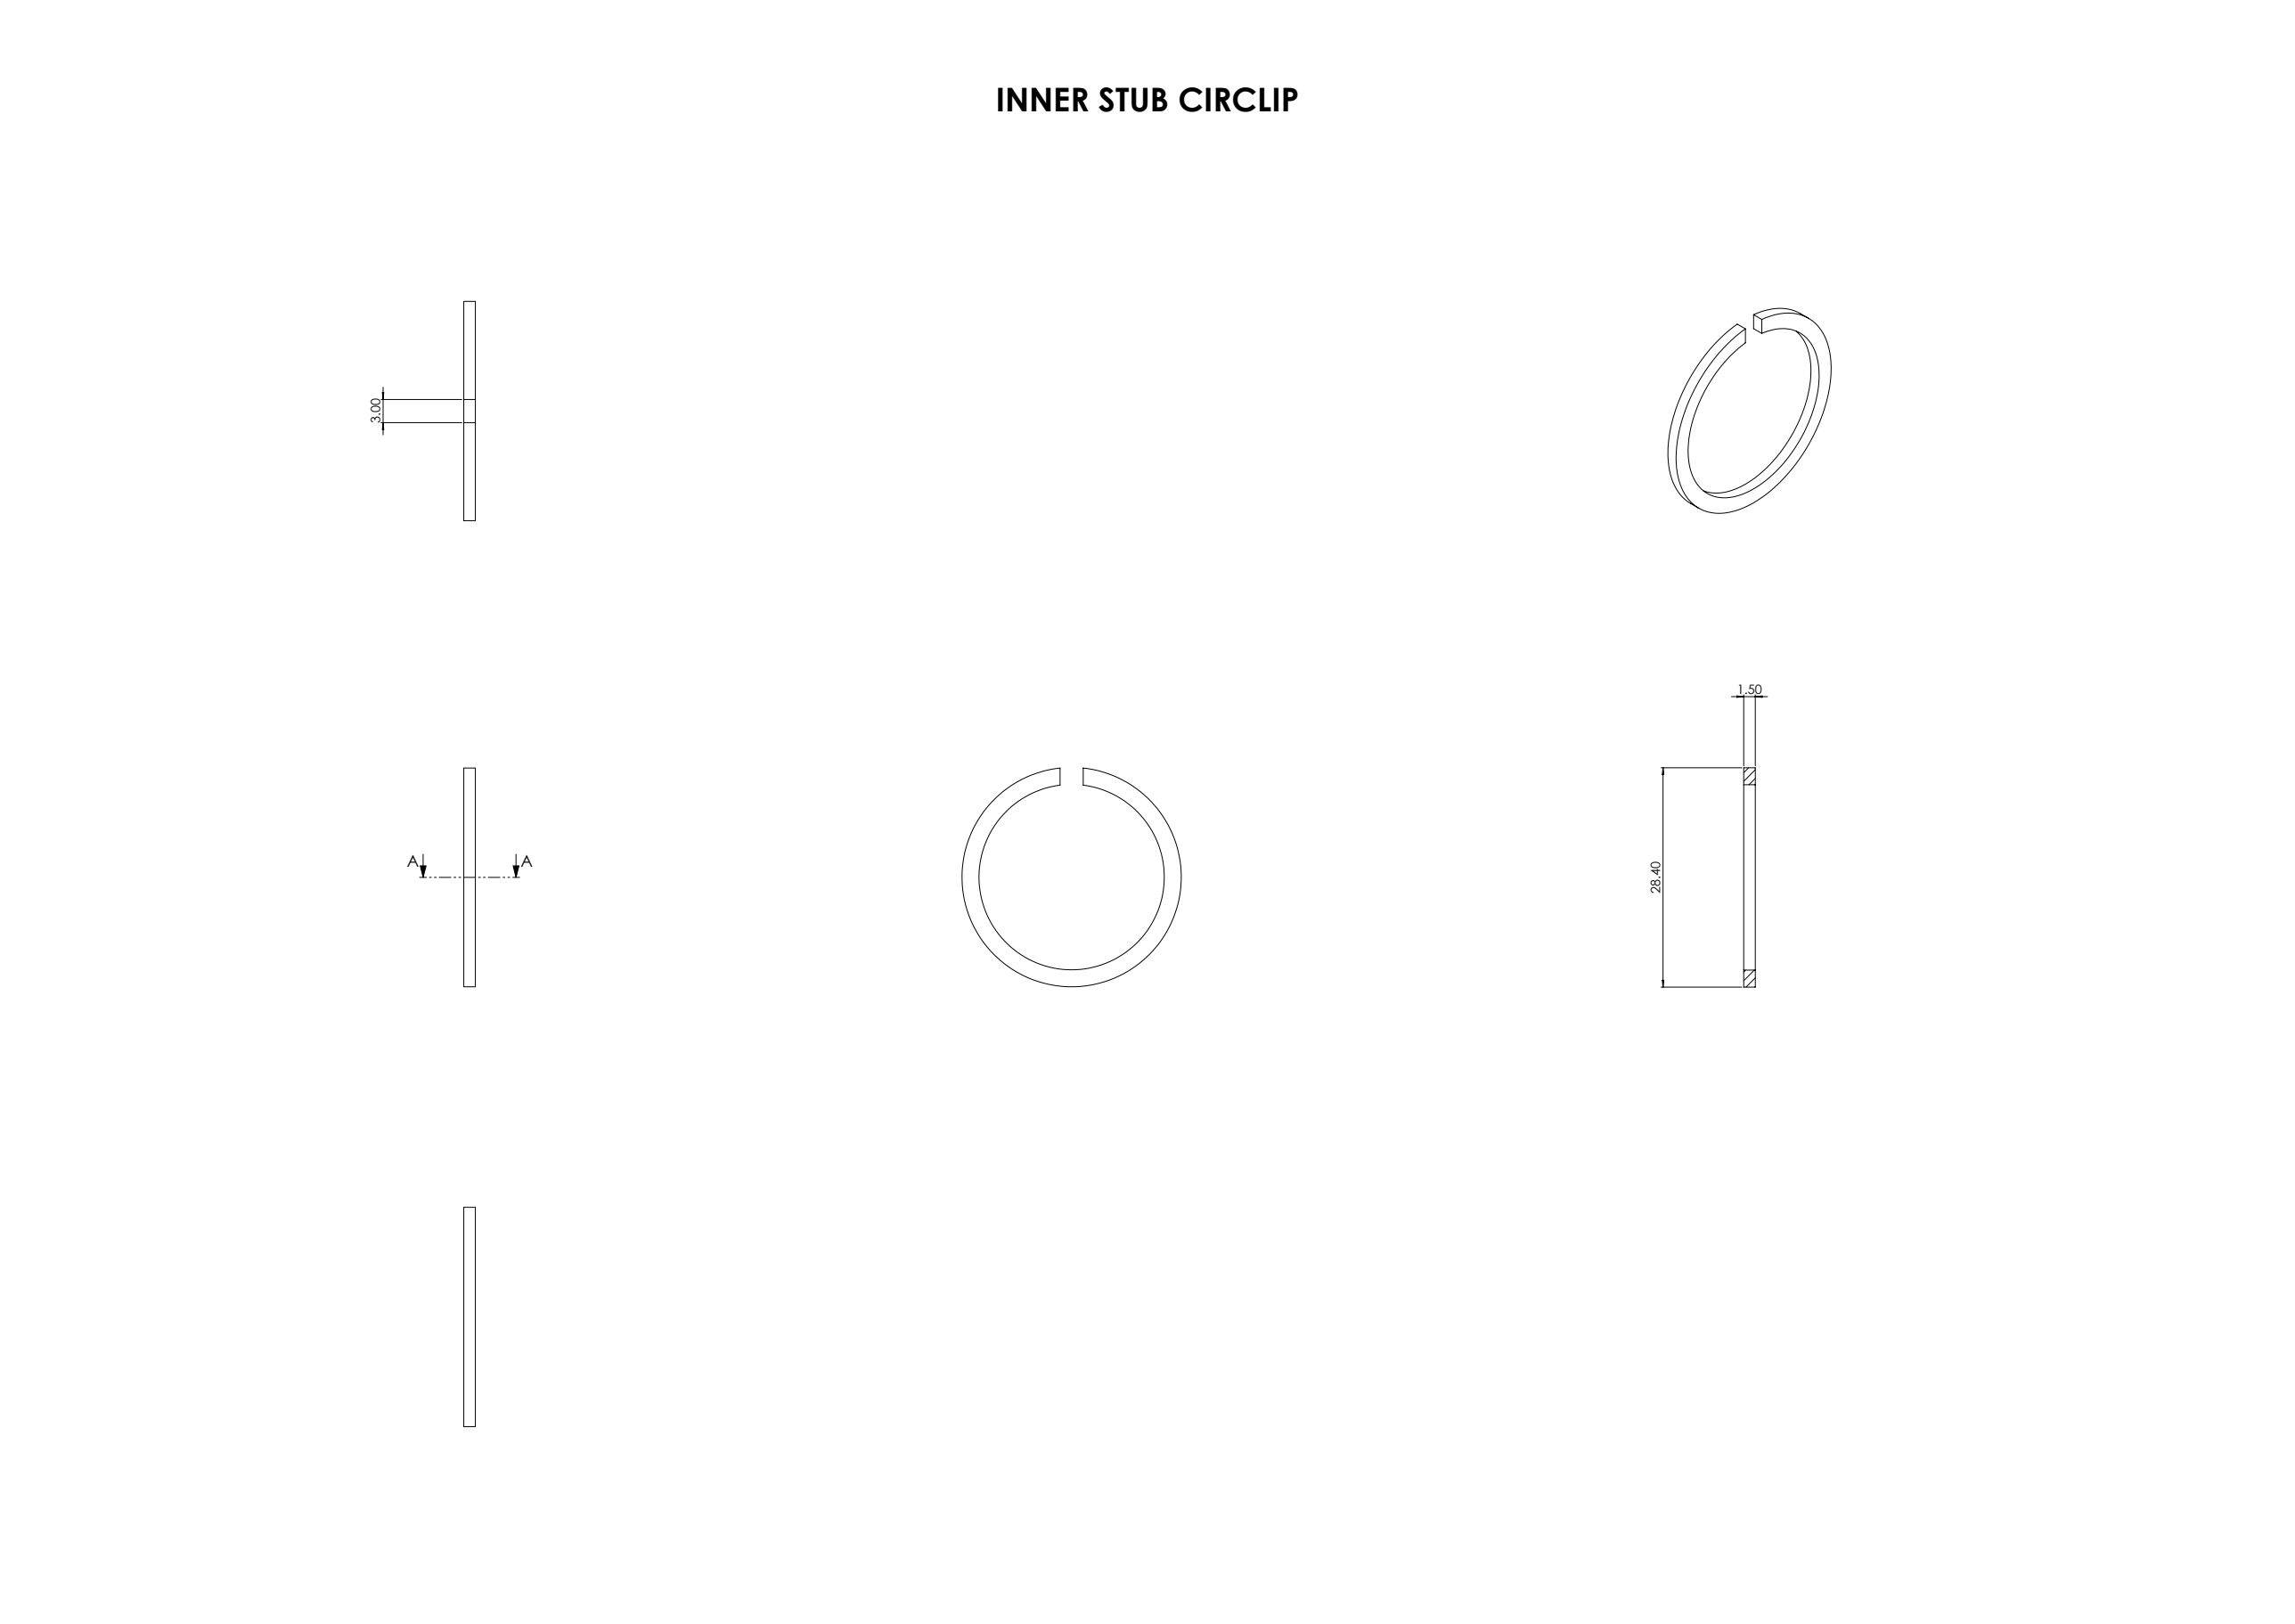
ISO-10303-21;
HEADER;
/* Generated by software containing ST-Developer
 * from STEP Tools, Inc. (www.steptools.com) 
 */

FILE_DESCRIPTION(
/* description */ (''),
/* implementation_level */ '2;1');

FILE_NAME(
/* name */ '17_Inner_Stub_Circlip.step',
/* time_stamp */ '2026-10-11T12:57:03-07:00',
/* author */ (''),
/* organization */ (''),
/* preprocessor_version */ 'ST-DEVELOPER v20.2',
/* originating_system */ 'Autodesk Translation Framework v15.15.0.0',
/* authorisation */ '');

FILE_SCHEMA (('AUTOMOTIVE_DESIGN { 1 0 10303 214 3 1 1 }'));
ENDSEC;

DATA;
#10=MECHANICAL_DESIGN_GEOMETRIC_PRESENTATION_REPRESENTATION('',(#272),#90374);
#238=SHAPE_REPRESENTATION_RELATIONSHIP('SRR','None',#90457,#255);
#255=ADVANCED_BREP_SHAPE_REPRESENTATION('',(#289),#90373);
#272=STYLED_ITEM('',(#90687),#289);
#289=MANIFOLD_SOLID_BREP('Body1',#40361);
#1824=PLANE('',#45261);
#1825=PLANE('',#45262);
#1826=PLANE('',#45263);
#1827=PLANE('',#45270);
#4536=FACE_OUTER_BOUND('',#7009,.T.);
#4537=FACE_OUTER_BOUND('',#7010,.T.);
#4538=FACE_OUTER_BOUND('',#7011,.T.);
#4539=FACE_OUTER_BOUND('',#7012,.T.);
#4540=FACE_OUTER_BOUND('',#7013,.T.);
#4541=FACE_OUTER_BOUND('',#7014,.T.);
#7009=EDGE_LOOP('',(#37203,#37204,#37205,#37206));
#7010=EDGE_LOOP('',(#37207,#37208,#37209,#37210));
#7011=EDGE_LOOP('',(#37211,#37212,#37213,#37214));
#7012=EDGE_LOOP('',(#37215,#37216,#37217,#37218));
#7013=EDGE_LOOP('',(#37219,#37220,#37221,#37222));
#7014=EDGE_LOOP('',(#37223,#37224,#37225,#37226));
#9420=CIRCLE('',#45264,14.2);
#9421=CIRCLE('',#45265,12.);
#9422=CIRCLE('',#45267,12.);
#9423=CIRCLE('',#45269,14.2);
#12844=LINE('',#90289,#15338);
#12845=LINE('',#90291,#15339);
#12846=LINE('',#90293,#15340);
#12847=LINE('',#90294,#15341);
#12848=LINE('',#90298,#15342);
#12849=LINE('',#90300,#15343);
#12850=LINE('',#90302,#15344);
#12851=LINE('',#90303,#15345);
#15338=VECTOR('',#57206,10.);
#15339=VECTOR('',#57207,10.);
#15340=VECTOR('',#57208,10.);
#15341=VECTOR('',#57209,10.);
#15342=VECTOR('',#57212,10.);
#15343=VECTOR('',#57213,10.);
#15344=VECTOR('',#57214,10.);
#15345=VECTOR('',#57215,10.);
#19066=VERTEX_POINT('',#90287);
#19067=VERTEX_POINT('',#90288);
#19068=VERTEX_POINT('',#90290);
#19069=VERTEX_POINT('',#90292);
#19070=VERTEX_POINT('',#90296);
#19071=VERTEX_POINT('',#90297);
#19072=VERTEX_POINT('',#90299);
#19073=VERTEX_POINT('',#90301);
#25113=EDGE_CURVE('',#19066,#19067,#12844,.T.);
#25114=EDGE_CURVE('',#19068,#19066,#12845,.T.);
#25115=EDGE_CURVE('',#19069,#19068,#12846,.T.);
#25116=EDGE_CURVE('',#19067,#19069,#12847,.T.);
#25117=EDGE_CURVE('',#19070,#19071,#12848,.T.);
#25118=EDGE_CURVE('',#19072,#19070,#12849,.T.);
#25119=EDGE_CURVE('',#19073,#19072,#12850,.T.);
#25120=EDGE_CURVE('',#19071,#19073,#12851,.T.);
#25121=EDGE_CURVE('',#19071,#19066,#9420,.T.);
#25122=EDGE_CURVE('',#19073,#19068,#9421,.T.);
#25123=EDGE_CURVE('',#19072,#19069,#9422,.T.);
#25124=EDGE_CURVE('',#19070,#19067,#9423,.T.);
#37203=ORIENTED_EDGE('',*,*,#25113,.F.);
#37204=ORIENTED_EDGE('',*,*,#25114,.F.);
#37205=ORIENTED_EDGE('',*,*,#25115,.F.);
#37206=ORIENTED_EDGE('',*,*,#25116,.F.);
#37207=ORIENTED_EDGE('',*,*,#25117,.F.);
#37208=ORIENTED_EDGE('',*,*,#25118,.F.);
#37209=ORIENTED_EDGE('',*,*,#25119,.F.);
#37210=ORIENTED_EDGE('',*,*,#25120,.F.);
#37211=ORIENTED_EDGE('',*,*,#25114,.T.);
#37212=ORIENTED_EDGE('',*,*,#25121,.F.);
#37213=ORIENTED_EDGE('',*,*,#25120,.T.);
#37214=ORIENTED_EDGE('',*,*,#25122,.T.);
#37215=ORIENTED_EDGE('',*,*,#25115,.T.);
#37216=ORIENTED_EDGE('',*,*,#25122,.F.);
#37217=ORIENTED_EDGE('',*,*,#25119,.T.);
#37218=ORIENTED_EDGE('',*,*,#25123,.T.);
#37219=ORIENTED_EDGE('',*,*,#25113,.T.);
#37220=ORIENTED_EDGE('',*,*,#25124,.F.);
#37221=ORIENTED_EDGE('',*,*,#25117,.T.);
#37222=ORIENTED_EDGE('',*,*,#25121,.T.);
#37223=ORIENTED_EDGE('',*,*,#25116,.T.);
#37224=ORIENTED_EDGE('',*,*,#25123,.F.);
#37225=ORIENTED_EDGE('',*,*,#25118,.T.);
#37226=ORIENTED_EDGE('',*,*,#25124,.T.);
#37946=CYLINDRICAL_SURFACE('',#45266,12.);
#37947=CYLINDRICAL_SURFACE('',#45268,14.2);
#40339=ADVANCED_FACE('',(#4536),#1824,.F.);
#40340=ADVANCED_FACE('',(#4537),#1825,.F.);
#40341=ADVANCED_FACE('',(#4538),#1826,.T.);
#40342=ADVANCED_FACE('',(#4539),#37946,.F.);
#40343=ADVANCED_FACE('',(#4540),#37947,.T.);
#40344=ADVANCED_FACE('',(#4541),#1827,.T.);
#40361=CLOSED_SHELL('',(#40339,#40340,#40341,#40342,#40343,#40344));
#45260=AXIS2_PLACEMENT_3D('',#90285,#57202,#57203);
#45261=AXIS2_PLACEMENT_3D('',#90286,#57204,#57205);
#45262=AXIS2_PLACEMENT_3D('',#90295,#57210,#57211);
#45263=AXIS2_PLACEMENT_3D('',#90304,#57216,#57217);
#45264=AXIS2_PLACEMENT_3D('',#90305,#57218,#57219);
#45265=AXIS2_PLACEMENT_3D('',#90306,#57220,#57221);
#45266=AXIS2_PLACEMENT_3D('',#90307,#57222,#57223);
#45267=AXIS2_PLACEMENT_3D('',#90308,#57224,#57225);
#45268=AXIS2_PLACEMENT_3D('',#90309,#57226,#57227);
#45269=AXIS2_PLACEMENT_3D('',#90310,#57228,#57229);
#45270=AXIS2_PLACEMENT_3D('',#90311,#57230,#57231);
#57202=DIRECTION('axis',(0.,0.,1.));
#57203=DIRECTION('refdir',(1.,0.,0.));
#57204=DIRECTION('center_axis',(0.,0.,-1.));
#57205=DIRECTION('ref_axis',(-1.,0.,0.));
#57206=DIRECTION('',(1.,0.,0.));
#57207=DIRECTION('',(0.,1.,0.));
#57208=DIRECTION('',(-1.,0.,0.));
#57209=DIRECTION('',(0.,-1.,0.));
#57210=DIRECTION('center_axis',(0.,0.,1.));
#57211=DIRECTION('ref_axis',(1.,0.,0.));
#57212=DIRECTION('',(-1.,0.,0.));
#57213=DIRECTION('',(0.,1.,0.));
#57214=DIRECTION('',(1.,0.,0.));
#57215=DIRECTION('',(0.,-1.,0.));
#57216=DIRECTION('center_axis',(-1.,0.,0.));
#57217=DIRECTION('ref_axis',(0.,0.,1.));
#57218=DIRECTION('center_axis',(1.,0.,0.));
#57219=DIRECTION('ref_axis',(0.,0.,-1.));
#57220=DIRECTION('center_axis',(1.,0.,0.));
#57221=DIRECTION('ref_axis',(0.,0.,-1.));
#57222=DIRECTION('center_axis',(1.,0.,0.));
#57223=DIRECTION('ref_axis',(0.,-1.,-1.22464679914735E-16));
#57224=DIRECTION('center_axis',(1.,0.,0.));
#57225=DIRECTION('ref_axis',(0.,0.,-1.));
#57226=DIRECTION('center_axis',(1.,0.,0.));
#57227=DIRECTION('ref_axis',(0.,-1.,-1.22464679914735E-16));
#57228=DIRECTION('center_axis',(1.,0.,0.));
#57229=DIRECTION('ref_axis',(0.,0.,-1.));
#57230=DIRECTION('center_axis',(1.,0.,0.));
#57231=DIRECTION('ref_axis',(0.,0.,-1.));
#90285=CARTESIAN_POINT('',(0.,0.,0.));
#90286=CARTESIAN_POINT('Origin',(668.75,13.,-1.5));
#90287=CARTESIAN_POINT('',(668.,14.1205523971267,-1.5));
#90288=CARTESIAN_POINT('',(669.5,14.1205523971267,-1.5));
#90289=CARTESIAN_POINT('',(668.75,14.1205523971267,-1.5));
#90290=CARTESIAN_POINT('',(668.,11.9058808997907,-1.5));
#90291=CARTESIAN_POINT('',(668.,13.6,-1.5));
#90292=CARTESIAN_POINT('',(669.5,11.9058808997907,-1.5));
#90293=CARTESIAN_POINT('',(668.75,11.9058808997907,-1.5));
#90294=CARTESIAN_POINT('',(669.5,12.5,-1.5));
#90295=CARTESIAN_POINT('Origin',(668.75,13.,1.5));
#90296=CARTESIAN_POINT('',(669.5,14.1205523971267,1.5));
#90297=CARTESIAN_POINT('',(668.,14.1205523971267,1.5));
#90298=CARTESIAN_POINT('',(668.75,14.1205523971267,1.5));
#90299=CARTESIAN_POINT('',(669.5,11.9058808997907,1.5));
#90300=CARTESIAN_POINT('',(669.5,12.5,1.5));
#90301=CARTESIAN_POINT('',(668.,11.9058808997907,1.5));
#90302=CARTESIAN_POINT('',(668.75,11.9058808997907,1.5));
#90303=CARTESIAN_POINT('',(668.,13.6,1.5));
#90304=CARTESIAN_POINT('Origin',(668.,14.2,0.));
#90305=CARTESIAN_POINT('Origin',(668.,0.,0.));
#90306=CARTESIAN_POINT('Origin',(668.,0.,0.));
#90307=CARTESIAN_POINT('Origin',(668.75,0.,0.));
#90308=CARTESIAN_POINT('Origin',(669.5,0.,0.));
#90309=CARTESIAN_POINT('Origin',(668.75,0.,0.));
#90310=CARTESIAN_POINT('Origin',(669.5,0.,0.));
#90311=CARTESIAN_POINT('Origin',(669.5,12.,0.));
#90354=UNCERTAINTY_MEASURE_WITH_UNIT(LENGTH_MEASURE(0.01),#90375,
'DISTANCE_ACCURACY_VALUE',
'Maximum model space distance between geometric entities at asserted c
onnectivities');
#90355=UNCERTAINTY_MEASURE_WITH_UNIT(LENGTH_MEASURE(0.01),#90375,
'DISTANCE_ACCURACY_VALUE',
'Maximum model space distance between geometric entities at asserted c
onnectivities');
#90373=(
GEOMETRIC_REPRESENTATION_CONTEXT(3)
GLOBAL_UNCERTAINTY_ASSIGNED_CONTEXT((#90354))
GLOBAL_UNIT_ASSIGNED_CONTEXT((#90375,#90377,#90378))
REPRESENTATION_CONTEXT('','3D')
);
#90374=(
GEOMETRIC_REPRESENTATION_CONTEXT(3)
GLOBAL_UNCERTAINTY_ASSIGNED_CONTEXT((#90355))
GLOBAL_UNIT_ASSIGNED_CONTEXT((#90375,#90377,#90378))
REPRESENTATION_CONTEXT('','3D')
);
#90375=(
LENGTH_UNIT()
NAMED_UNIT(*)
SI_UNIT(.MILLI.,.METRE.)
);
#90377=(
NAMED_UNIT(*)
PLANE_ANGLE_UNIT()
SI_UNIT($,.RADIAN.)
);
#90378=(
NAMED_UNIT(*)
SI_UNIT($,.STERADIAN.)
SOLID_ANGLE_UNIT()
);
#90396=SHAPE_DEFINITION_REPRESENTATION(#90414,#90457);
#90414=PRODUCT_DEFINITION_SHAPE('',$,#90476);
#90457=SHAPE_REPRESENTATION('',(#45260),#90373);
#90458=PRODUCT_DEFINITION_CONTEXT('part definition',#90514,'design');
#90476=PRODUCT_DEFINITION('2026-10-11-12-53-16-624',
'17_Inner_Stub_Circlip',#90494,#90458);
#90494=PRODUCT_DEFINITION_FORMATION('',$,#90533);
#90514=APPLICATION_CONTEXT(
'Core Data for Automotive Mechanical Design Process');
#90515=PRODUCT_CONTEXT('part definition',#90514,'mechanical');
#90533=PRODUCT('2026-10-11-12-53-16-624','17_Inner_Stub_Circlip',$,(#90515));
#90681=COLOUR_RGB('Grey',0.48,0.52,0.57);
#90682=FILL_AREA_STYLE_COLOUR('',#90681);
#90683=FILL_AREA_STYLE('',(#90682));
#90684=SURFACE_STYLE_FILL_AREA(#90683);
#90685=SURFACE_SIDE_STYLE('',(#90684));
#90686=SURFACE_STYLE_USAGE(.BOTH.,#90685);
#90687=PRESENTATION_STYLE_ASSIGNMENT((#90686));
ENDSEC;
END-ISO-10303-21;
